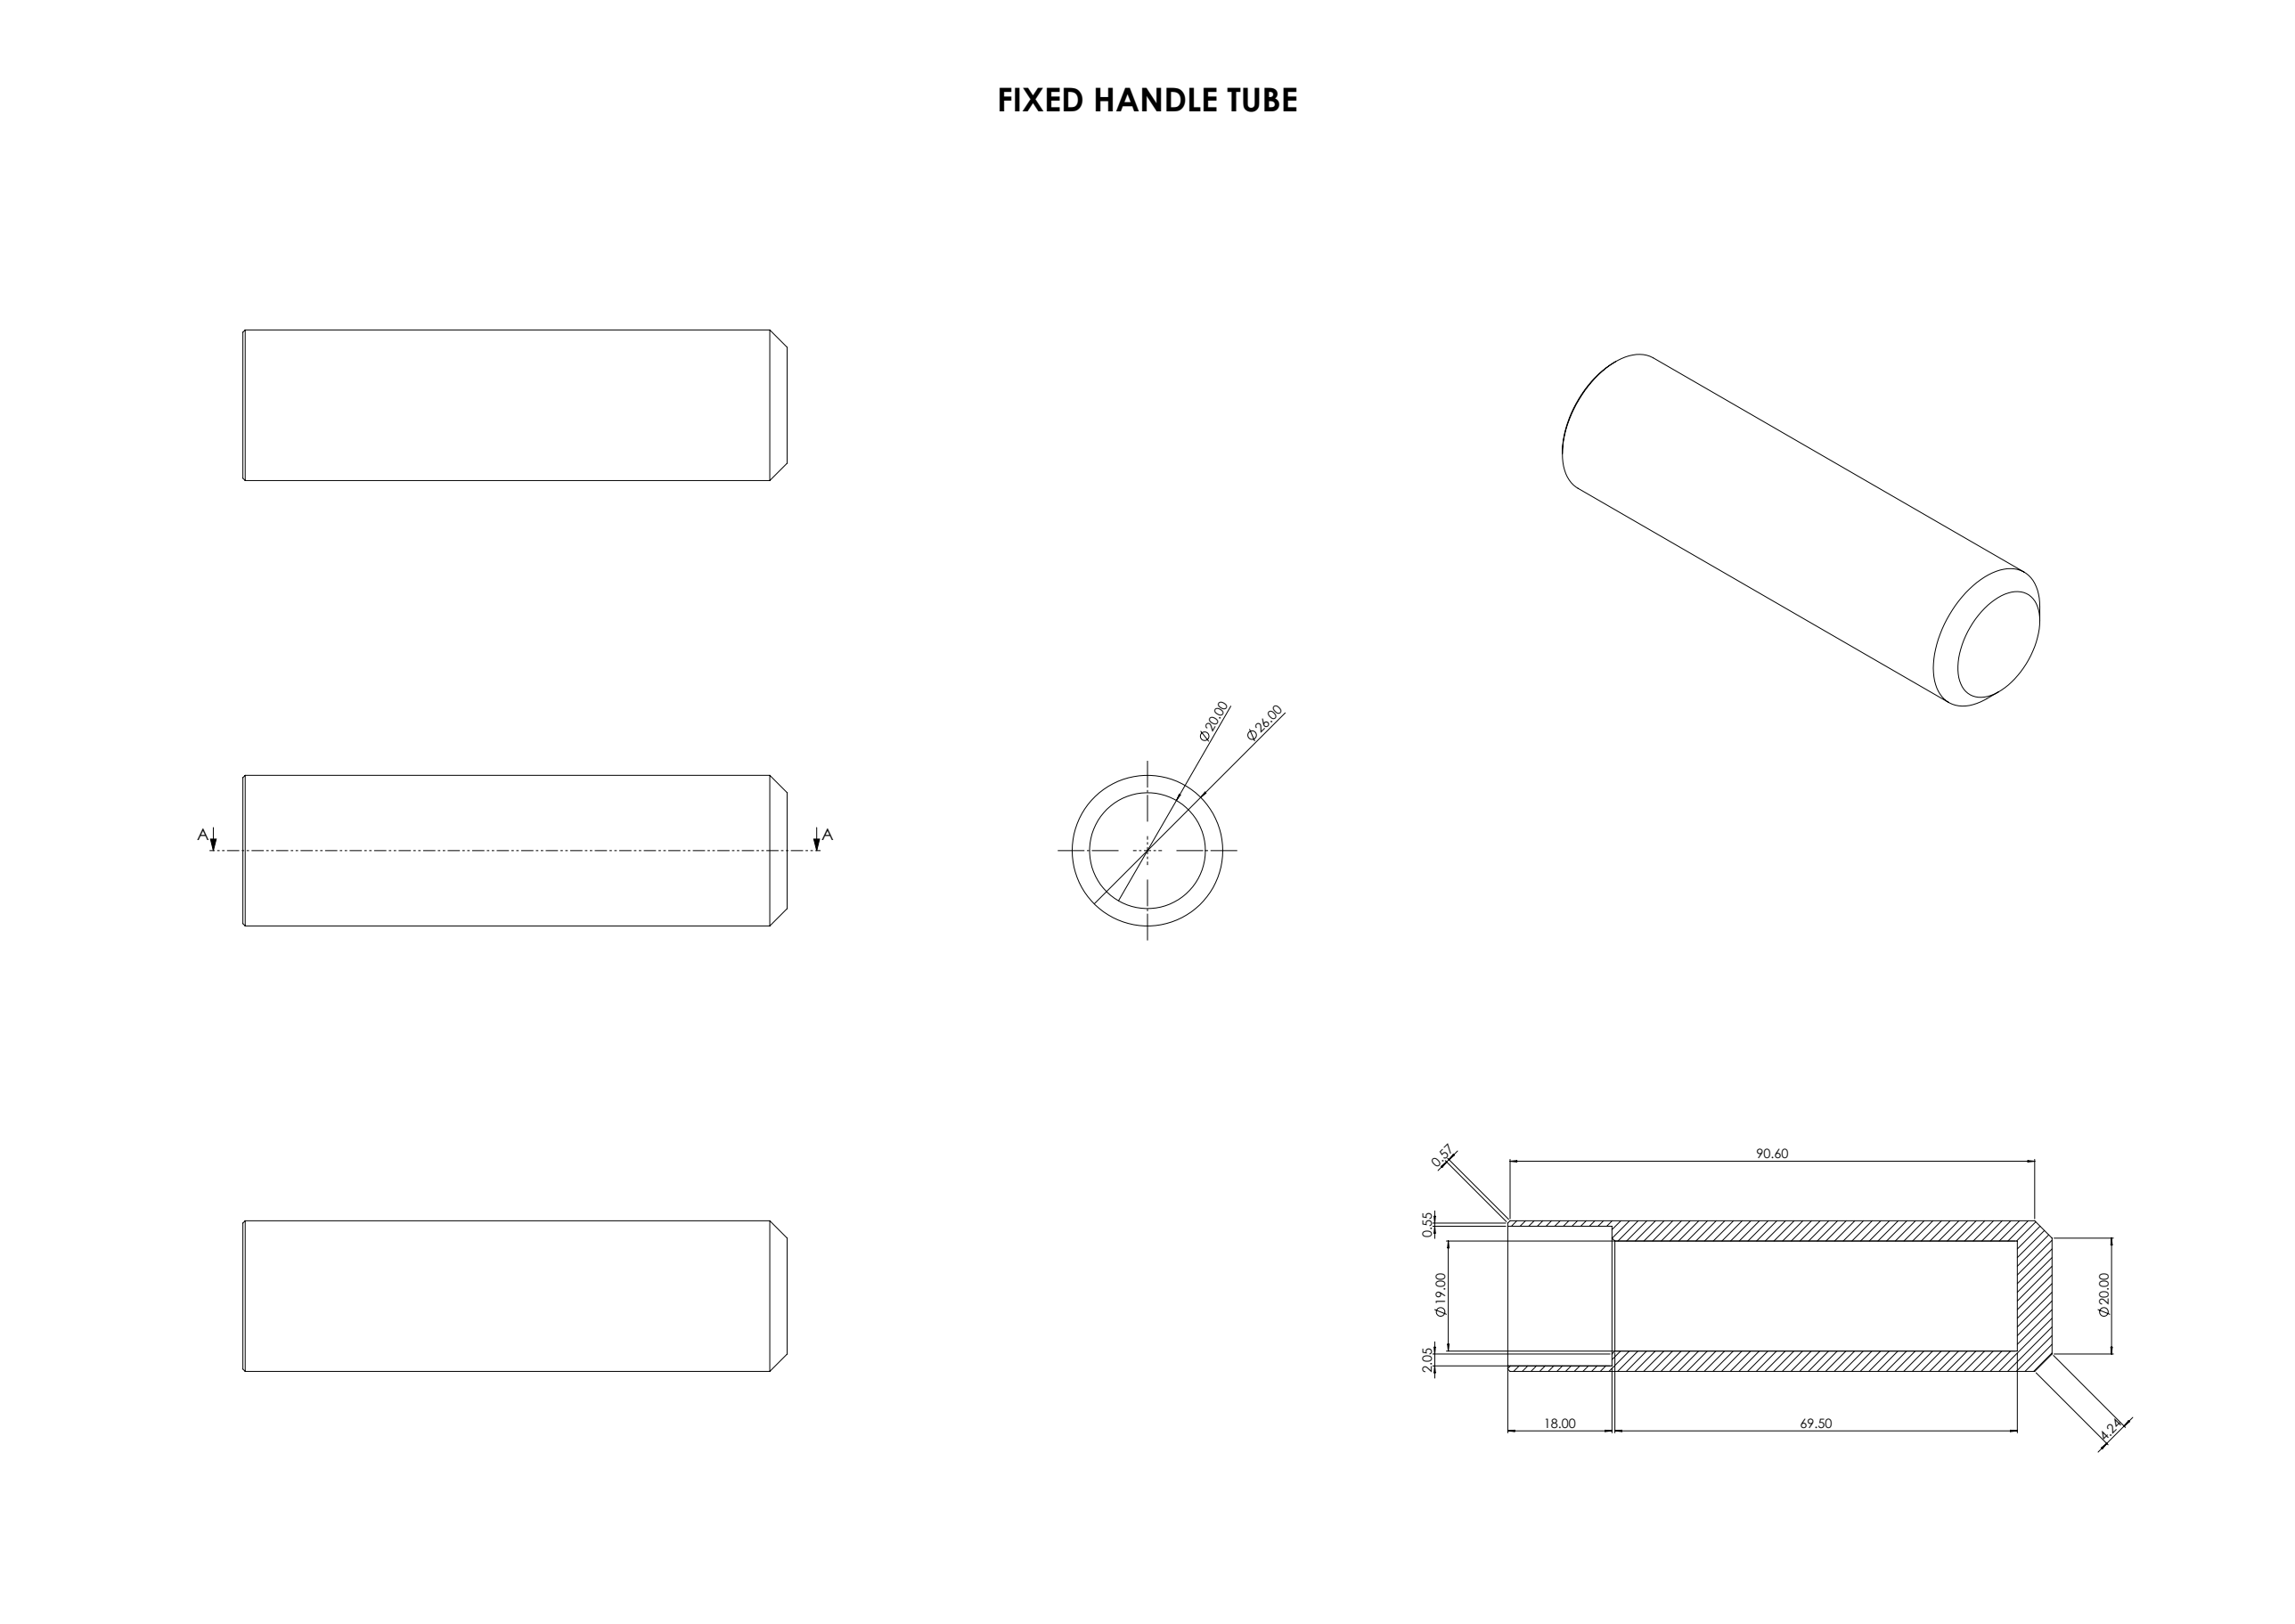
ISO-10303-21;
HEADER;
/* Generated by software containing ST-Developer
 * from STEP Tools, Inc. (www.steptools.com) 
 */

FILE_DESCRIPTION(
/* description */ (''),
/* implementation_level */ '2;1');

FILE_NAME(
/* name */ '18_Fixed_Handle_Tube.step',
/* time_stamp */ '2026-10-26T03:55:20-07:00',
/* author */ (''),
/* organization */ (''),
/* preprocessor_version */ 'ST-DEVELOPER v20.2',
/* originating_system */ 'Autodesk Translation Framework v15.15.0.0',
/* authorisation */ '');

FILE_SCHEMA (('AUTOMOTIVE_DESIGN { 1 0 10303 214 3 1 1 }'));
ENDSEC;

DATA;
#10=MECHANICAL_DESIGN_GEOMETRIC_PRESENTATION_REPRESENTATION('',(#186),#45236);
#146=SHAPE_REPRESENTATION_RELATIONSHIP('SRR','None',#45325,#166);
#166=ADVANCED_BREP_SHAPE_REPRESENTATION('',(#206),#45227);
#186=STYLED_ITEM('',(#45477),#206);
#206=MANIFOLD_SOLID_BREP('Body1',#16528);
#1001=FACE_BOUND('',#3456,.T.);
#1002=FACE_BOUND('',#3459,.T.);
#1329=PLANE('',#17558);
#1330=PLANE('',#17562);
#1331=PLANE('',#17570);
#1332=PLANE('',#17571);
#1747=CYLINDRICAL_SURFACE('',#17556,9.5);
#1748=CYLINDRICAL_SURFACE('',#17560,12.05);
#1749=CYLINDRICAL_SURFACE('',#17566,13.);
#2417=FACE_OUTER_BOUND('',#3453,.T.);
#2418=FACE_OUTER_BOUND('',#3454,.T.);
#2419=FACE_OUTER_BOUND('',#3455,.T.);
#2420=FACE_OUTER_BOUND('',#3457,.T.);
#2421=FACE_OUTER_BOUND('',#3458,.T.);
#2422=FACE_OUTER_BOUND('',#3460,.T.);
#2423=FACE_OUTER_BOUND('',#3461,.T.);
#2424=FACE_OUTER_BOUND('',#3462,.T.);
#2425=FACE_OUTER_BOUND('',#3463,.T.);
#2426=FACE_OUTER_BOUND('',#3464,.T.);
#3453=EDGE_LOOP('',(#13768,#13769,#13770,#13771,#13772));
#3454=EDGE_LOOP('',(#13773,#13774,#13775,#13776,#13777));
#3455=EDGE_LOOP('',(#13778));
#3456=EDGE_LOOP('',(#13779));
#3457=EDGE_LOOP('',(#13780,#13781,#13782,#13783));
#3458=EDGE_LOOP('',(#13784));
#3459=EDGE_LOOP('',(#13785));
#3460=EDGE_LOOP('',(#13786,#13787,#13788,#13789));
#3461=EDGE_LOOP('',(#13790,#13791,#13792,#13793));
#3462=EDGE_LOOP('',(#13794,#13795,#13796,#13797));
#3463=EDGE_LOOP('',(#13798));
#3464=EDGE_LOOP('',(#13799));
#4661=LINE('',#40553,#5972);
#4662=LINE('',#40560,#5973);
#4663=LINE('',#40566,#5974);
#4664=LINE('',#40574,#5975);
#4665=LINE('',#40578,#5976);
#4666=LINE('',#40582,#5977);
#5972=VECTOR('',#20490,9.75);
#5973=VECTOR('',#20499,9.5);
#5974=VECTOR('',#20506,12.05);
#5975=VECTOR('',#20517,12.8);
#5976=VECTOR('',#20522,13.);
#5977=VECTOR('',#20527,11.5);
#6774=CIRCLE('',#17553,10.);
#6775=CIRCLE('',#17554,9.5);
#6776=CIRCLE('',#17555,9.5);
#6777=CIRCLE('',#17557,9.5);
#6778=CIRCLE('',#17559,12.05);
#6779=CIRCLE('',#17561,12.05);
#6780=CIRCLE('',#17563,12.6);
#6781=CIRCLE('',#17565,13.);
#6782=CIRCLE('',#17567,13.);
#6783=CIRCLE('',#17569,10.);
#7916=VERTEX_POINT('',#40550);
#7917=VERTEX_POINT('',#40552);
#7918=VERTEX_POINT('',#40554);
#7919=VERTEX_POINT('',#40558);
#7920=VERTEX_POINT('',#40562);
#7921=VERTEX_POINT('',#40565);
#7922=VERTEX_POINT('',#40569);
#7923=VERTEX_POINT('',#40572);
#7924=VERTEX_POINT('',#40576);
#7925=VERTEX_POINT('',#40580);
#9947=EDGE_CURVE('',#7916,#7916,#6774,.T.);
#9948=EDGE_CURVE('',#7916,#7917,#4661,.T.);
#9949=EDGE_CURVE('',#7917,#7918,#6775,.T.);
#9950=EDGE_CURVE('',#7918,#7917,#6776,.T.);
#9951=EDGE_CURVE('',#7919,#7919,#6777,.T.);
#9952=EDGE_CURVE('',#7919,#7918,#4662,.T.);
#9953=EDGE_CURVE('',#7920,#7920,#6778,.T.);
#9954=EDGE_CURVE('',#7920,#7921,#4663,.T.);
#9955=EDGE_CURVE('',#7921,#7921,#6779,.T.);
#9956=EDGE_CURVE('',#7922,#7922,#6780,.T.);
#9957=EDGE_CURVE('',#7923,#7923,#6781,.T.);
#9958=EDGE_CURVE('',#7923,#7922,#4664,.T.);
#9959=EDGE_CURVE('',#7924,#7924,#6782,.T.);
#9960=EDGE_CURVE('',#7924,#7923,#4665,.T.);
#9961=EDGE_CURVE('',#7925,#7925,#6783,.T.);
#9962=EDGE_CURVE('',#7925,#7924,#4666,.T.);
#13768=ORIENTED_EDGE('',*,*,#9947,.T.);
#13769=ORIENTED_EDGE('',*,*,#9948,.T.);
#13770=ORIENTED_EDGE('',*,*,#9949,.T.);
#13771=ORIENTED_EDGE('',*,*,#9950,.T.);
#13772=ORIENTED_EDGE('',*,*,#9948,.F.);
#13773=ORIENTED_EDGE('',*,*,#9951,.T.);
#13774=ORIENTED_EDGE('',*,*,#9952,.T.);
#13775=ORIENTED_EDGE('',*,*,#9949,.F.);
#13776=ORIENTED_EDGE('',*,*,#9950,.F.);
#13777=ORIENTED_EDGE('',*,*,#9952,.F.);
#13778=ORIENTED_EDGE('',*,*,#9953,.F.);
#13779=ORIENTED_EDGE('',*,*,#9947,.F.);
#13780=ORIENTED_EDGE('',*,*,#9953,.T.);
#13781=ORIENTED_EDGE('',*,*,#9954,.T.);
#13782=ORIENTED_EDGE('',*,*,#9955,.F.);
#13783=ORIENTED_EDGE('',*,*,#9954,.F.);
#13784=ORIENTED_EDGE('',*,*,#9956,.F.);
#13785=ORIENTED_EDGE('',*,*,#9955,.T.);
#13786=ORIENTED_EDGE('',*,*,#9957,.F.);
#13787=ORIENTED_EDGE('',*,*,#9958,.T.);
#13788=ORIENTED_EDGE('',*,*,#9956,.T.);
#13789=ORIENTED_EDGE('',*,*,#9958,.F.);
#13790=ORIENTED_EDGE('',*,*,#9959,.F.);
#13791=ORIENTED_EDGE('',*,*,#9960,.T.);
#13792=ORIENTED_EDGE('',*,*,#9957,.T.);
#13793=ORIENTED_EDGE('',*,*,#9960,.F.);
#13794=ORIENTED_EDGE('',*,*,#9961,.F.);
#13795=ORIENTED_EDGE('',*,*,#9962,.T.);
#13796=ORIENTED_EDGE('',*,*,#9959,.T.);
#13797=ORIENTED_EDGE('',*,*,#9962,.F.);
#13798=ORIENTED_EDGE('',*,*,#9961,.T.);
#13799=ORIENTED_EDGE('',*,*,#9951,.F.);
#15511=CONICAL_SURFACE('',#17552,9.75,0.785398163397442);
#15512=CONICAL_SURFACE('',#17564,12.8,0.785398163397459);
#15513=CONICAL_SURFACE('',#17568,11.5,0.785398163397447);
#16145=ADVANCED_FACE('',(#2417),#15511,.F.);
#16146=ADVANCED_FACE('',(#2418),#1747,.F.);
#16147=ADVANCED_FACE('',(#2419,#1001),#1329,.T.);
#16148=ADVANCED_FACE('',(#2420),#1748,.F.);
#16149=ADVANCED_FACE('',(#2421,#1002),#1330,.T.);
#16150=ADVANCED_FACE('',(#2422),#15512,.T.);
#16151=ADVANCED_FACE('',(#2423),#1749,.T.);
#16152=ADVANCED_FACE('',(#2424),#15513,.T.);
#16153=ADVANCED_FACE('',(#2425),#1331,.T.);
#16154=ADVANCED_FACE('',(#2426),#1332,.T.);
#16528=CLOSED_SHELL('',(#16145,#16146,#16147,#16148,#16149,#16150,#16151,
#16152,#16153,#16154));
#17551=AXIS2_PLACEMENT_3D('',#40548,#20484,#20485);
#17552=AXIS2_PLACEMENT_3D('',#40549,#20486,#20487);
#17553=AXIS2_PLACEMENT_3D('',#40551,#20488,#20489);
#17554=AXIS2_PLACEMENT_3D('',#40555,#20491,#20492);
#17555=AXIS2_PLACEMENT_3D('',#40556,#20493,#20494);
#17556=AXIS2_PLACEMENT_3D('',#40557,#20495,#20496);
#17557=AXIS2_PLACEMENT_3D('',#40559,#20497,#20498);
#17558=AXIS2_PLACEMENT_3D('',#40561,#20500,#20501);
#17559=AXIS2_PLACEMENT_3D('',#40563,#20502,#20503);
#17560=AXIS2_PLACEMENT_3D('',#40564,#20504,#20505);
#17561=AXIS2_PLACEMENT_3D('',#40567,#20507,#20508);
#17562=AXIS2_PLACEMENT_3D('',#40568,#20509,#20510);
#17563=AXIS2_PLACEMENT_3D('',#40570,#20511,#20512);
#17564=AXIS2_PLACEMENT_3D('',#40571,#20513,#20514);
#17565=AXIS2_PLACEMENT_3D('',#40573,#20515,#20516);
#17566=AXIS2_PLACEMENT_3D('',#40575,#20518,#20519);
#17567=AXIS2_PLACEMENT_3D('',#40577,#20520,#20521);
#17568=AXIS2_PLACEMENT_3D('',#40579,#20523,#20524);
#17569=AXIS2_PLACEMENT_3D('',#40581,#20525,#20526);
#17570=AXIS2_PLACEMENT_3D('',#40583,#20528,#20529);
#17571=AXIS2_PLACEMENT_3D('',#40584,#20530,#20531);
#20484=DIRECTION('axis',(0.,0.,1.));
#20485=DIRECTION('refdir',(1.,0.,0.));
#20486=DIRECTION('center_axis',(-1.,0.,0.));
#20487=DIRECTION('ref_axis',(0.,-1.,0.));
#20488=DIRECTION('center_axis',(-1.,0.,0.));
#20489=DIRECTION('ref_axis',(0.,-1.,0.));
#20490=DIRECTION('',(0.707106781186552,-0.707106781186543,8.65956056235488E-17));
#20491=DIRECTION('center_axis',(1.,0.,0.));
#20492=DIRECTION('ref_axis',(0.,-1.,0.));
#20493=DIRECTION('center_axis',(1.,0.,0.));
#20494=DIRECTION('ref_axis',(0.,-1.,0.));
#20495=DIRECTION('center_axis',(1.,0.,0.));
#20496=DIRECTION('ref_axis',(0.,1.,0.));
#20497=DIRECTION('center_axis',(1.,0.,0.));
#20498=DIRECTION('ref_axis',(0.,0.,-1.));
#20499=DIRECTION('',(-1.,0.,0.));
#20500=DIRECTION('center_axis',(-1.,0.,0.));
#20501=DIRECTION('ref_axis',(0.,0.,1.));
#20502=DIRECTION('center_axis',(1.,0.,0.));
#20503=DIRECTION('ref_axis',(0.,0.,-1.));
#20504=DIRECTION('center_axis',(1.,0.,0.));
#20505=DIRECTION('ref_axis',(0.,1.,0.));
#20506=DIRECTION('',(-1.,0.,0.));
#20507=DIRECTION('center_axis',(1.,0.,0.));
#20508=DIRECTION('ref_axis',(0.,0.,-1.));
#20509=DIRECTION('center_axis',(-1.,0.,0.));
#20510=DIRECTION('ref_axis',(0.,0.,1.));
#20511=DIRECTION('center_axis',(1.,0.,0.));
#20512=DIRECTION('ref_axis',(0.,0.,-1.));
#20513=DIRECTION('center_axis',(1.,0.,0.));
#20514=DIRECTION('ref_axis',(0.,1.,0.));
#20515=DIRECTION('center_axis',(1.,0.,0.));
#20516=DIRECTION('ref_axis',(0.,0.,-1.));
#20517=DIRECTION('',(-0.70710678118654,0.707106781186555,8.65956056235503E-17));
#20518=DIRECTION('center_axis',(1.,0.,0.));
#20519=DIRECTION('ref_axis',(0.,1.,0.));
#20520=DIRECTION('center_axis',(1.,0.,0.));
#20521=DIRECTION('ref_axis',(0.,0.,-1.));
#20522=DIRECTION('',(-1.,0.,0.));
#20523=DIRECTION('center_axis',(-1.,0.,0.));
#20524=DIRECTION('ref_axis',(0.,1.,0.));
#20525=DIRECTION('center_axis',(1.,0.,0.));
#20526=DIRECTION('ref_axis',(0.,0.,-1.));
#20527=DIRECTION('',(-0.707106781186548,-0.707106781186547,-8.65956056235492E-17));
#20528=DIRECTION('center_axis',(1.,0.,0.));
#20529=DIRECTION('ref_axis',(0.,0.,-1.));
#20530=DIRECTION('center_axis',(-1.,0.,0.));
#20531=DIRECTION('ref_axis',(0.,0.,1.));
#40548=CARTESIAN_POINT('',(0.,0.,0.));
#40549=CARTESIAN_POINT('Origin',(224.25,0.,0.));
#40550=CARTESIAN_POINT('',(224.,10.,-1.22464679914735E-15));
#40551=CARTESIAN_POINT('Origin',(224.,0.,0.));
#40552=CARTESIAN_POINT('',(224.5,9.5,1.16341445918999E-15));
#40553=CARTESIAN_POINT('',(224.25,9.75,-1.19403062916867E-15));
#40554=CARTESIAN_POINT('',(224.5,-9.5,-1.16341445918999E-15));
#40555=CARTESIAN_POINT('Origin',(224.5,0.,0.));
#40556=CARTESIAN_POINT('Origin',(224.5,0.,0.));
#40557=CARTESIAN_POINT('Origin',(259.,0.,0.));
#40558=CARTESIAN_POINT('',(294.,-9.5,-1.16341445918999E-15));
#40559=CARTESIAN_POINT('Origin',(294.,0.,0.));
#40560=CARTESIAN_POINT('',(259.,-9.5,-1.16341445918999E-15));
#40561=CARTESIAN_POINT('Origin',(224.,12.05,0.));
#40562=CARTESIAN_POINT('',(224.,-12.05,-1.47569939297256E-15));
#40563=CARTESIAN_POINT('Origin',(224.,0.,0.));
#40564=CARTESIAN_POINT('Origin',(215.,0.,0.));
#40565=CARTESIAN_POINT('',(206.,-12.05,-1.47569939297256E-15));
#40566=CARTESIAN_POINT('',(215.,-12.05,-1.47569939297256E-15));
#40567=CARTESIAN_POINT('Origin',(206.,0.,0.));
#40568=CARTESIAN_POINT('Origin',(206.,12.6,0.));
#40569=CARTESIAN_POINT('',(206.,-12.6,-1.54305496692566E-15));
#40570=CARTESIAN_POINT('Origin',(206.,0.,0.));
#40571=CARTESIAN_POINT('Origin',(206.2,0.,0.));
#40572=CARTESIAN_POINT('',(206.4,-13.,-1.59204083889156E-15));
#40573=CARTESIAN_POINT('Origin',(206.4,0.,0.));
#40574=CARTESIAN_POINT('',(206.2,-12.8,-1.56754790290861E-15));
#40575=CARTESIAN_POINT('Origin',(251.7,0.,0.));
#40576=CARTESIAN_POINT('',(297.,-13.,-1.59204083889156E-15));
#40577=CARTESIAN_POINT('Origin',(297.,0.,0.));
#40578=CARTESIAN_POINT('',(251.7,-13.,-1.59204083889156E-15));
#40579=CARTESIAN_POINT('Origin',(298.5,0.,0.));
#40580=CARTESIAN_POINT('',(300.,-10.,-1.22464679914735E-15));
#40581=CARTESIAN_POINT('Origin',(300.,0.,0.));
#40582=CARTESIAN_POINT('',(298.5,-11.5,-1.40834381901946E-15));
#40583=CARTESIAN_POINT('Origin',(300.,0.,0.));
#40584=CARTESIAN_POINT('Origin',(294.,9.5,0.));
#45205=UNCERTAINTY_MEASURE_WITH_UNIT(LENGTH_MEASURE(0.01),#45237,
'DISTANCE_ACCURACY_VALUE',
'Maximum model space distance between geometric entities at asserted c
onnectivities');
#45214=UNCERTAINTY_MEASURE_WITH_UNIT(LENGTH_MEASURE(0.01),#45237,
'DISTANCE_ACCURACY_VALUE',
'Maximum model space distance between geometric entities at asserted c
onnectivities');
#45227=(
GEOMETRIC_REPRESENTATION_CONTEXT(3)
GLOBAL_UNCERTAINTY_ASSIGNED_CONTEXT((#45205))
GLOBAL_UNIT_ASSIGNED_CONTEXT((#45237,#45239,#45240))
REPRESENTATION_CONTEXT('','3D')
);
#45236=(
GEOMETRIC_REPRESENTATION_CONTEXT(3)
GLOBAL_UNCERTAINTY_ASSIGNED_CONTEXT((#45214))
GLOBAL_UNIT_ASSIGNED_CONTEXT((#45237,#45239,#45240))
REPRESENTATION_CONTEXT('','3D')
);
#45237=(
LENGTH_UNIT()
NAMED_UNIT(*)
SI_UNIT(.MILLI.,.METRE.)
);
#45239=(
NAMED_UNIT(*)
PLANE_ANGLE_UNIT()
SI_UNIT($,.RADIAN.)
);
#45240=(
NAMED_UNIT(*)
SI_UNIT($,.STERADIAN.)
SOLID_ANGLE_UNIT()
);
#45253=SHAPE_DEFINITION_REPRESENTATION(#45274,#45325);
#45274=PRODUCT_DEFINITION_SHAPE('',$,#45347);
#45325=SHAPE_REPRESENTATION('',(#17551),#45227);
#45334=PRODUCT_DEFINITION_CONTEXT('part definition',#45399,'design');
#45347=PRODUCT_DEFINITION('2026-10-25-23-38-28-911',
'18_Fixed_Handle_Tube',#45368,#45334);
#45368=PRODUCT_DEFINITION_FORMATION('',$,#45413);
#45399=APPLICATION_CONTEXT(
'Core Data for Automotive Mechanical Design Process');
#45400=PRODUCT_CONTEXT('part definition',#45399,'mechanical');
#45413=PRODUCT('2026-10-25-23-38-28-911','18_Fixed_Handle_Tube',$,(#45400));
#45471=COLOUR_RGB('Sky Blue',0.24,0.69,0.87);
#45472=FILL_AREA_STYLE_COLOUR('',#45471);
#45473=FILL_AREA_STYLE('',(#45472));
#45474=SURFACE_STYLE_FILL_AREA(#45473);
#45475=SURFACE_SIDE_STYLE('',(#45474));
#45476=SURFACE_STYLE_USAGE(.BOTH.,#45475);
#45477=PRESENTATION_STYLE_ASSIGNMENT((#45476));
ENDSEC;
END-ISO-10303-21;
